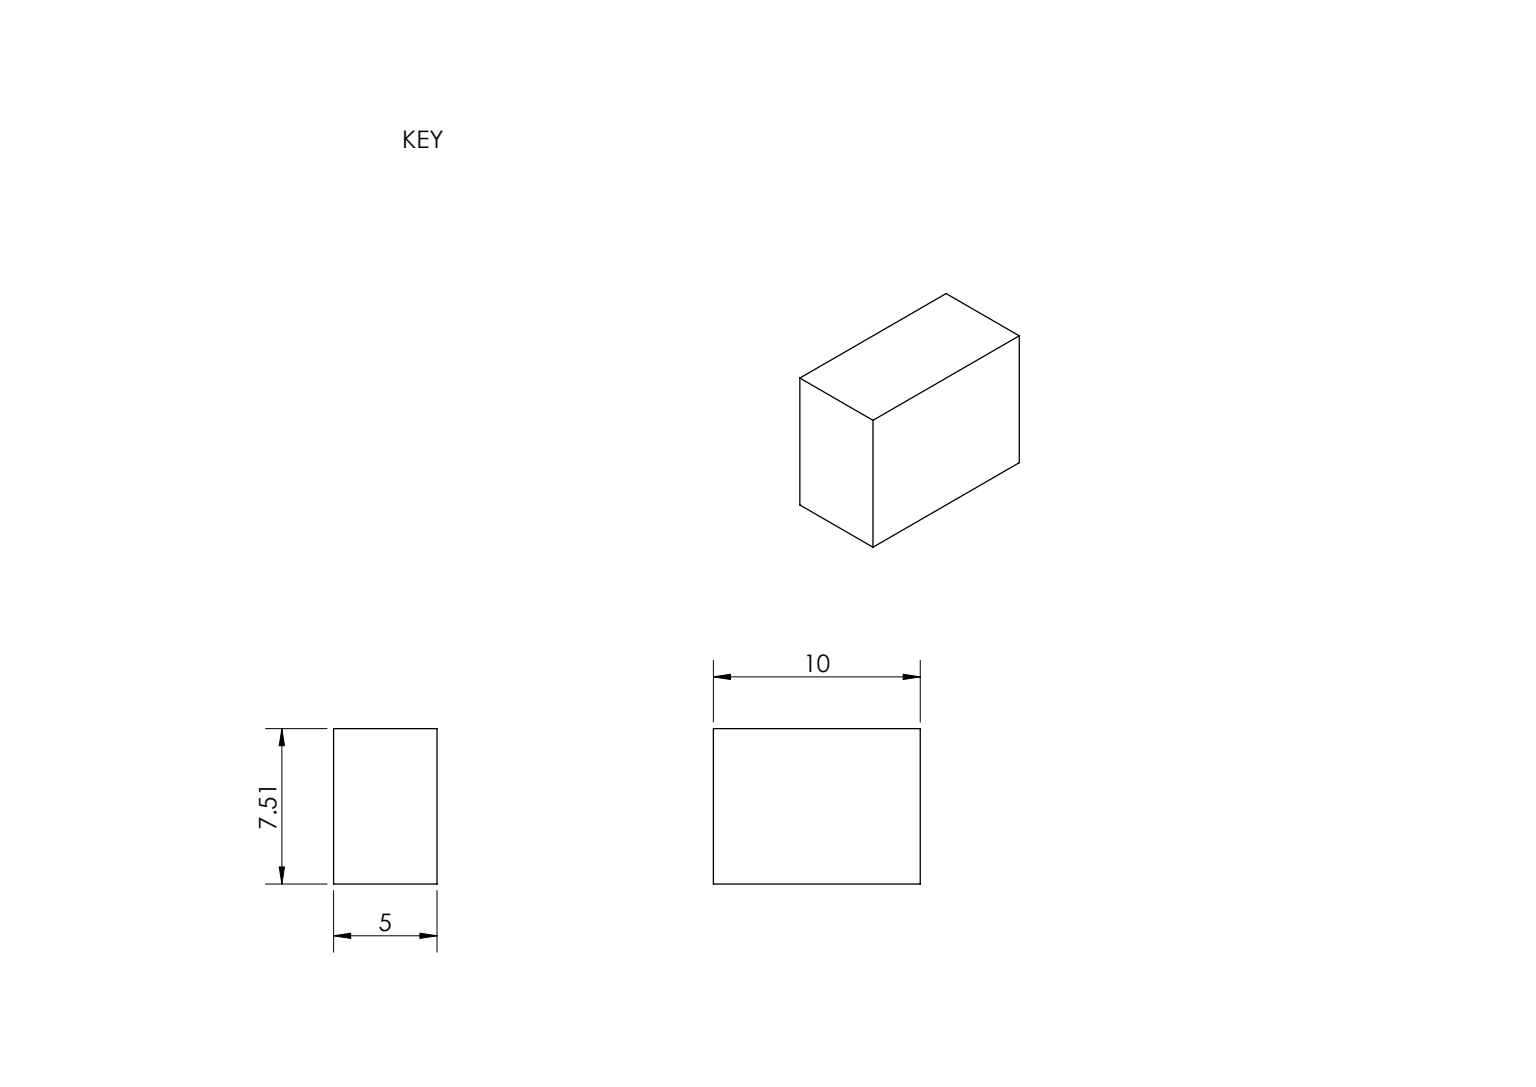
ISO-10303-21;
HEADER;
FILE_DESCRIPTION (('STEP AP214'),
    '1' );
FILE_NAME ('key.step',
    '2026-10-08T09:53:37',
    ( '' ),
    ( '' ),
    'SwSTEP 2.0',
    'SolidWorks 2026',
    '' );
FILE_SCHEMA (( 'AUTOMOTIVE_DESIGN' ));
ENDSEC;

DATA;
#19=AXIS2_PLACEMENT_3D ( 'NONE', #55225, #15366, #9737 ) ;
#383=( GEOMETRIC_REPRESENTATION_CONTEXT ( 3 ) GLOBAL_UNCERTAINTY_ASSIGNED_CONTEXT ( ( #16132 ) ) GLOBAL_UNIT_ASSIGNED_CONTEXT ( ( #58527, #47619, #18304 ) ) REPRESENTATION_CONTEXT ( 'NONE', 'WORKASPACE' ) );
#670=PLANE ( 'NONE',  #22865 ) ;
#687=ORIENTED_EDGE ( 'NONE', *, *, #21533, .F. ) ;
#692=SURFACE_SIDE_STYLE ('',( #30321 ) ) ;
#695=PLANE ( 'NONE',  #20980 ) ;
#1023=DIRECTION ( 'NONE',  ( 0.000000000000000000, -1.000000000000000000, 0.000000000000000000 ) ) ;
#1746=DIRECTION ( 'NONE',  ( -1.000000000000000000, -0.000000000000000000, -0.000000000000000000 ) ) ;
#2167=EDGE_CURVE ( 'NONE', #37724, #39945, #55632, .T. ) ;
#2801=DIRECTION ( 'NONE',  ( 0.000000000000000000, 1.000000000000000000, 0.000000000000000000 ) ) ;
#3898=VECTOR ( 'NONE', #1746, 1000.000000000000000 ) ;
#3952=MECHANICAL_DESIGN_GEOMETRIC_PRESENTATION_REPRESENTATION('',(#71150),#383);
#4204=( LENGTH_UNIT ( ) NAMED_UNIT ( * ) SI_UNIT ( .MILLI., .METRE. ) );
#4518=EDGE_CURVE ( 'NONE', #39945, #5325, #48483, .T. ) ;
#4952=SURFACE_SIDE_STYLE ('',( #9080 ) ) ;
#5325=VERTEX_POINT ( 'NONE', #24542 ) ;
#6306=( NAMED_UNIT ( * ) SI_UNIT ( $, .STERADIAN. ) SOLID_ANGLE_UNIT ( ) );
#6406=PRODUCT_DEFINITION_FORMATION_WITH_SPECIFIED_SOURCE ( 'ANY', '', #48755, .NOT_KNOWN. ) ;
#6637=FACE_OUTER_BOUND ( 'NONE', #63194, .T. ) ;
#6650=CARTESIAN_POINT ( 'NONE',  ( -2.499999999999997780, 8.494897427831771708, -19.01812422950394676 ) ) ;
#6662=SURFACE_STYLE_USAGE ( .BOTH. , #692 ) ;
#6695=VERTEX_POINT ( 'NONE', #45004 ) ;
#8097=DIRECTION ( 'NONE',  ( 0.000000000000000000, -0.000000000000000000, -1.000000000000000000 ) ) ;
#9080=SURFACE_STYLE_FILL_AREA ( #72225 ) ;
#9224=EDGE_CURVE ( 'NONE', #34982, #38545, #28058, .T. ) ;
#9388=CARTESIAN_POINT ( 'NONE',  ( -2.500000000000000000, 16.00000000000000000, 0.000000000000000000 ) ) ;
#9609=EDGE_CURVE ( 'NONE', #5325, #55639, #73082, .T. ) ;
#9737=DIRECTION ( 'NONE',  ( 2.889240119132116694E-16, -1.000000000000000000, 0.000000000000000000 ) ) ;
#9969=APPLICATION_CONTEXT ( 'automotive_design' ) ;
#10321=CARTESIAN_POINT ( 'NONE',  ( -2.500000000000000000, 16.00000000000000000, -10.00000000000000178 ) ) ;
#11069=EDGE_CURVE ( 'NONE', #6695, #34982, #20563, .T. ) ;
#11908=LINE ( 'NONE', #6650, #41232 ) ;
#11959=ORIENTED_EDGE ( 'NONE', *, *, #63581, .T. ) ;
#12006=DIRECTION ( 'NONE',  ( -0.000000000000000000, 0.000000000000000000, 1.000000000000000000 ) ) ;
#14915=DIRECTION ( 'NONE',  ( 5.778480238264233142E-17, -1.000000000000000000, 0.000000000000000000 ) ) ;
#14998=FACE_OUTER_BOUND ( 'NONE', #61959, .T. ) ;
#15064=ORIENTED_EDGE ( 'NONE', *, *, #72245, .F. ) ;
#15098=ORIENTED_EDGE ( 'NONE', *, *, #11069, .T. ) ;
#15366=DIRECTION ( 'NONE',  ( -1.000000000000000000, -2.889240119132116694E-16, 0.000000000000000000 ) ) ;
#15700=EDGE_CURVE ( 'NONE', #38545, #39945, #11908, .T. ) ;
#16132=UNCERTAINTY_MEASURE_WITH_UNIT (LENGTH_MEASURE( 1.000000000000000082E-05 ), #58527, 'distance_accuracy_value', 'NONE');
#16180=LINE ( 'NONE', #21069, #61063 ) ;
#16797=CARTESIAN_POINT ( 'NONE',  ( -2.499999999999997780, 8.494897427831771708, -10.00000000000000178 ) ) ;
#17069=ORIENTED_EDGE ( 'NONE', *, *, #36059, .T. ) ;
#17917=DIRECTION ( 'NONE',  ( 1.000000000000000000, 5.778480238264233142E-17, -0.000000000000000000 ) ) ;
#17942=FILL_AREA_STYLE_COLOUR ( '', #26671 ) ;
#18292=CARTESIAN_POINT ( 'NONE',  ( -2.499999999999997780, 8.494897427831771708, -10.00000000000000178 ) ) ;
#18304=( NAMED_UNIT ( * ) SI_UNIT ( $, .STERADIAN. ) SOLID_ANGLE_UNIT ( ) );
#18325=LINE ( 'NONE', #52532, #45553 ) ;
#18875=DIRECTION ( 'NONE',  ( 0.000000000000000000, 0.000000000000000000, 1.000000000000000000 ) ) ;
#19089=DIRECTION ( 'NONE',  ( 0.000000000000000000, 0.000000000000000000, 1.000000000000000000 ) ) ;
#19252=CARTESIAN_POINT ( 'NONE',  ( 2.500000000000000000, 16.00000000000000000, -19.01812422950394676 ) ) ;
#19415=ADVANCED_FACE ( 'NONE', ( #45123 ), #28926, .T. ) ;
#19713=EDGE_LOOP ( 'NONE', ( #45893, #58178, #43286, #25168 ) ) ;
#19735=DIRECTION ( 'NONE',  ( 1.000000000000000000, 0.000000000000000000, 0.000000000000000000 ) ) ;
#20563=LINE ( 'NONE', #54042, #32379 ) ;
#20980=AXIS2_PLACEMENT_3D ( 'NONE', #23585, #23963, #69442 ) ;
#21069=CARTESIAN_POINT ( 'NONE',  ( -2.500000000000000000, 16.00000000000000000, -10.00000000000000178 ) ) ;
#21087=SURFACE_STYLE_USAGE ( .BOTH. , #4952 ) ;
#21154=PRODUCT_DEFINITION_SHAPE ( 'NONE', 'NONE',  #40301 ) ;
#21533=EDGE_CURVE ( 'NONE', #55639, #37724, #40538, .T. ) ;
#22865=AXIS2_PLACEMENT_3D ( 'NONE', #23558, #17917, #40861 ) ;
#23457=SHAPE_REPRESENTATION ( 'key', ( #43395 ), #59100 ) ;
#23558=CARTESIAN_POINT ( 'NONE',  ( 2.500000000000000000, 16.00000000000000000, -19.01812422950394676 ) ) ;
#23585=CARTESIAN_POINT ( 'NONE',  ( -1.066668064568189757E-15, -1.540743955509788682E-30, -10.00000000000000178 ) ) ;
#23963=DIRECTION ( 'NONE',  ( 0.000000000000000000, 0.000000000000000000, 1.000000000000000000 ) ) ;
#24542=CARTESIAN_POINT ( 'NONE',  ( 2.500000000000000444, 8.494897427831771708, 0.000000000000000000 ) ) ;
#24637=ORIENTED_EDGE ( 'NONE', *, *, #4518, .F. ) ;
#25168=ORIENTED_EDGE ( 'NONE', *, *, #21533, .T. ) ;
#25559=ADVANCED_FACE ( 'NONE', ( #57806 ), #695, .F. ) ;
#26299=( GEOMETRIC_REPRESENTATION_CONTEXT ( 3 ) GLOBAL_UNCERTAINTY_ASSIGNED_CONTEXT ( ( #43771 ) ) GLOBAL_UNIT_ASSIGNED_CONTEXT ( ( #4204, #50028, #27096 ) ) REPRESENTATION_CONTEXT ( 'NONE', 'WORKASPACE' ) );
#26312=DIRECTION ( 'NONE',  ( 2.889240119132116694E-16, -1.000000000000000000, 0.000000000000000000 ) ) ;
#26611=VECTOR ( 'NONE', #65778, 1000.000000000000000 ) ;
#26671=COLOUR_RGB ( '', 0.66274510, 0.83137255, 0.94901961) ;
#27096=( NAMED_UNIT ( * ) SI_UNIT ( $, .STERADIAN. ) SOLID_ANGLE_UNIT ( ) );
#27153=ORIENTED_EDGE ( 'NONE', *, *, #11069, .F. ) ;
#28058=LINE ( 'NONE', #16797, #52879 ) ;
#28545=CARTESIAN_POINT ( 'NONE',  ( 0.000000000000000000, 0.000000000000000000, 0.000000000000000000 ) ) ;
#28600=CARTESIAN_POINT ( 'NONE',  ( 2.500000000000000000, 16.00000000000000000, 0.000000000000000000 ) ) ;
#28926=PLANE ( 'NONE',  #49773 ) ;
#29703=ADVANCED_FACE ( 'NONE', ( #29908 ), #48322, .T. ) ;
#29908=FACE_OUTER_BOUND ( 'NONE', #35122, .T. ) ;
#30321=SURFACE_STYLE_FILL_AREA ( #52147 ) ;
#30386=VECTOR ( 'NONE', #19089, 1000.000000000000000 ) ;
#30580=PLANE ( 'NONE',  #43045 ) ;
#31609=CARTESIAN_POINT ( 'NONE',  ( -2.499999999999997780, 8.494897427831771708, 0.000000000000000000 ) ) ;
#32283=PLANE ( 'NONE',  #19 ) ;
#32379=VECTOR ( 'NONE', #14915, 1000.000000000000000 ) ;
#32504=ADVANCED_FACE ( 'NONE', ( #66299 ), #30580, .T. ) ;
#33333=ORIENTED_EDGE ( 'NONE', *, *, #2167, .F. ) ;
#34866=( NAMED_UNIT ( * ) PLANE_ANGLE_UNIT ( ) SI_UNIT ( $, .RADIAN. ) );
#34982=VERTEX_POINT ( 'NONE', #65531 ) ;
#35122=EDGE_LOOP ( 'NONE', ( #69723, #38672, #24637, #71523 ) ) ;
#35908=STYLED_ITEM ( 'NONE', ( #45160 ), #63624 ) ;
#36059=EDGE_CURVE ( 'NONE', #38545, #50675, #57683, .T. ) ;
#36243=EDGE_LOOP ( 'NONE', ( #69673, #54921, #687, #38370 ) ) ;
#37724=VERTEX_POINT ( 'NONE', #68878 ) ;
#37754=UNCERTAINTY_MEASURE_WITH_UNIT (LENGTH_MEASURE( 1.000000000000000082E-05 ), #47260, 'distance_accuracy_value', 'NONE');
#38370=ORIENTED_EDGE ( 'NONE', *, *, #63581, .F. ) ;
#38545=VERTEX_POINT ( 'NONE', #18292 ) ;
#38672=ORIENTED_EDGE ( 'NONE', *, *, #72245, .T. ) ;
#39643=CARTESIAN_POINT ( 'NONE',  ( -2.500000000000000000, 16.00000000000000000, -10.00000000000000178 ) ) ;
#39829=VECTOR ( 'NONE', #26312, 1000.000000000000000 ) ;
#39945=VERTEX_POINT ( 'NONE', #31609 ) ;
#39953=EDGE_CURVE ( 'NONE', #50675, #6695, #16180, .T. ) ;
#40301=PRODUCT_DEFINITION ( 'UNKNOWN', '', #6406, #54422 ) ;
#40538=LINE ( 'NONE', #63485, #3898 ) ;
#40737=APPLICATION_CONTEXT ( 'automotive_design' ) ;
#40849=CARTESIAN_POINT ( 'NONE',  ( -2.499999999999997780, 8.494897427831771708, -19.01812422950394676 ) ) ;
#40861=DIRECTION ( 'NONE',  ( -5.778480238264233142E-17, 1.000000000000000000, 0.000000000000000000 ) ) ;
#41232=VECTOR ( 'NONE', #63809, 1000.000000000000000 ) ;
#41608=SHAPE_REPRESENTATION_RELATIONSHIP ( 'NONE' , 'NONE' ,  #23457, #55235 ) ;
#42783=CLOSED_SHELL ( 'NONE', ( #64028, #32504, #45108, #29703, #19415, #25559 ) ) ;
#43045=AXIS2_PLACEMENT_3D ( 'NONE', #60657, #2801, #60295 ) ;
#43286=ORIENTED_EDGE ( 'NONE', *, *, #9609, .T. ) ;
#43395=AXIS2_PLACEMENT_3D ( 'NONE', #48320, #71232, #19735 ) ;
#43661=DIRECTION ( 'NONE',  ( 1.000000000000000000, 0.000000000000000000, 0.000000000000000000 ) ) ;
#43703=ORIENTED_EDGE ( 'NONE', *, *, #15700, .T. ) ;
#43771=UNCERTAINTY_MEASURE_WITH_UNIT (LENGTH_MEASURE( 1.000000000000000082E-05 ), #4204, 'distance_accuracy_value', 'NONE');
#45004=CARTESIAN_POINT ( 'NONE',  ( 2.500000000000000000, 16.00000000000000000, -10.00000000000000178 ) ) ;
#45108=ADVANCED_FACE ( 'NONE', ( #6637 ), #670, .T. ) ;
#45123=FACE_OUTER_BOUND ( 'NONE', #19713, .T. ) ;
#45160=PRESENTATION_STYLE_ASSIGNMENT (( #21087 ) ) ;
#45553=VECTOR ( 'NONE', #59295, 1000.000000000000000 ) ;
#45666=DIRECTION ( 'NONE',  ( -5.778480238264233142E-17, 1.000000000000000000, -0.000000000000000000 ) ) ;
#45671=DIRECTION ( 'NONE',  ( -2.889240119132116694E-16, 1.000000000000000000, 0.000000000000000000 ) ) ;
#45877=DIRECTION ( 'NONE',  ( 1.000000000000000000, 0.000000000000000000, 0.000000000000000000 ) ) ;
#45893=ORIENTED_EDGE ( 'NONE', *, *, #2167, .T. ) ;
#47055=VECTOR ( 'NONE', #45671, 1000.000000000000000 ) ;
#47260=( LENGTH_UNIT ( ) NAMED_UNIT ( * ) SI_UNIT ( .MILLI., .METRE. ) );
#47619=( NAMED_UNIT ( * ) PLANE_ANGLE_UNIT ( ) SI_UNIT ( $, .RADIAN. ) );
#47937=COLOUR_RGB ( '', 0.66274510, 0.83137255, 0.94901961) ;
#48320=CARTESIAN_POINT ( 'NONE',  ( 0.000000000000000000, 0.000000000000000000, 0.000000000000000000 ) ) ;
#48322=PLANE ( 'NONE',  #69402 ) ;
#48483=LINE ( 'NONE', #71398, #26611 ) ;
#48755=PRODUCT ( 'key', 'key', '', ( #66680 ) ) ;
#48963=ORIENTED_EDGE ( 'NONE', *, *, #56177, .F. ) ;
#49108=MECHANICAL_DESIGN_GEOMETRIC_PRESENTATION_REPRESENTATION('',(#35908),#26299);
#49773=AXIS2_PLACEMENT_3D ( 'NONE', #28545, #12006, #45877 ) ;
#50028=( NAMED_UNIT ( * ) PLANE_ANGLE_UNIT ( ) SI_UNIT ( $, .RADIAN. ) );
#50253=VECTOR ( 'NONE', #45666, 1000.000000000000000 ) ;
#50675=VERTEX_POINT ( 'NONE', #39643 ) ;
#52147=FILL_AREA_STYLE ('',( #17942 ) ) ;
#52532=CARTESIAN_POINT ( 'NONE',  ( 2.500000000000000444, 8.494897427831771708, -19.01812422950394676 ) ) ;
#52879=VECTOR ( 'NONE', #63402, 1000.000000000000000 ) ;
#53676=LINE ( 'NONE', #59695, #30386 ) ;
#54042=CARTESIAN_POINT ( 'NONE',  ( 2.500000000000000000, 16.00000000000000000, -10.00000000000000178 ) ) ;
#54422=PRODUCT_DEFINITION_CONTEXT ( 'detailed design', #40737, 'design' ) ;
#54921=ORIENTED_EDGE ( 'NONE', *, *, #56177, .T. ) ;
#55225=CARTESIAN_POINT ( 'NONE',  ( -2.500000000000000000, 16.00000000000000000, -19.01812422950394676 ) ) ;
#55235=ADVANCED_BREP_SHAPE_REPRESENTATION ( '', ( #63624, #43395 ), #59100 ) ;
#55632=LINE ( 'NONE', #9388, #39829 ) ;
#55639=VERTEX_POINT ( 'NONE', #28600 ) ;
#56177=EDGE_CURVE ( 'NONE', #50675, #37724, #53676, .T. ) ;
#56182=CARTESIAN_POINT ( 'NONE',  ( 2.500000000000000000, 16.00000000000000000, 0.000000000000000000 ) ) ;
#56891=SHAPE_DEFINITION_REPRESENTATION ( #21154, #23457 ) ;
#57328=ORIENTED_EDGE ( 'NONE', *, *, #39953, .T. ) ;
#57683=LINE ( 'NONE', #10321, #47055 ) ;
#57806=FACE_OUTER_BOUND ( 'NONE', #65461, .T. ) ;
#58178=ORIENTED_EDGE ( 'NONE', *, *, #4518, .T. ) ;
#58527=( LENGTH_UNIT ( ) NAMED_UNIT ( * ) SI_UNIT ( .MILLI., .METRE. ) );
#59100=( GEOMETRIC_REPRESENTATION_CONTEXT ( 3 ) GLOBAL_UNCERTAINTY_ASSIGNED_CONTEXT ( ( #37754 ) ) GLOBAL_UNIT_ASSIGNED_CONTEXT ( ( #47260, #34866, #6306 ) ) REPRESENTATION_CONTEXT ( 'NONE', 'WORKASPACE' ) );
#59295=DIRECTION ( 'NONE',  ( 0.000000000000000000, 0.000000000000000000, 1.000000000000000000 ) ) ;
#59339=ORIENTED_EDGE ( 'NONE', *, *, #36059, .F. ) ;
#59695=CARTESIAN_POINT ( 'NONE',  ( -2.500000000000000000, 16.00000000000000000, -19.01812422950394676 ) ) ;
#59843=ORIENTED_EDGE ( 'NONE', *, *, #9609, .F. ) ;
#60295=DIRECTION ( 'NONE',  ( 0.000000000000000000, -0.000000000000000000, 1.000000000000000000 ) ) ;
#60657=CARTESIAN_POINT ( 'NONE',  ( -2.500000000000000000, 16.00000000000000000, -19.01812422950394676 ) ) ;
#61063=VECTOR ( 'NONE', #43661, 1000.000000000000000 ) ;
#61959=EDGE_LOOP ( 'NONE', ( #59339, #43703, #33333, #48963 ) ) ;
#63194=EDGE_LOOP ( 'NONE', ( #27153, #11959, #59843, #15064 ) ) ;
#63402=DIRECTION ( 'NONE',  ( -1.000000000000000000, 0.000000000000000000, 0.000000000000000000 ) ) ;
#63485=CARTESIAN_POINT ( 'NONE',  ( -2.500000000000000000, 16.00000000000000000, 0.000000000000000000 ) ) ;
#63581=EDGE_CURVE ( 'NONE', #6695, #55639, #71849, .T. ) ;
#63624=MANIFOLD_SOLID_BREP ( 'Boss-Extrude1', #42783 ) ;
#63809=DIRECTION ( 'NONE',  ( 0.000000000000000000, 0.000000000000000000, 1.000000000000000000 ) ) ;
#64028=ADVANCED_FACE ( 'NONE', ( #14998 ), #32283, .T. ) ;
#64928=PRESENTATION_STYLE_ASSIGNMENT (( #6662 ) ) ;
#65461=EDGE_LOOP ( 'NONE', ( #17069, #57328, #15098, #70522 ) ) ;
#65531=CARTESIAN_POINT ( 'NONE',  ( 2.500000000000000444, 8.494897427831771708, -10.00000000000000178 ) ) ;
#65778=DIRECTION ( 'NONE',  ( 1.000000000000000000, 0.000000000000000000, 0.000000000000000000 ) ) ;
#66299=FACE_OUTER_BOUND ( 'NONE', #36243, .T. ) ;
#66680=PRODUCT_CONTEXT ( 'NONE', #9969, 'mechanical' ) ;
#67145=VECTOR ( 'NONE', #18875, 1000.000000000000000 ) ;
#67713=FILL_AREA_STYLE_COLOUR ( '', #47937 ) ;
#68878=CARTESIAN_POINT ( 'NONE',  ( -2.500000000000000000, 16.00000000000000000, 0.000000000000000000 ) ) ;
#69402=AXIS2_PLACEMENT_3D ( 'NONE', #40849, #1023, #8097 ) ;
#69442=DIRECTION ( 'NONE',  ( 1.000000000000000000, 0.000000000000000000, 0.000000000000000000 ) ) ;
#69673=ORIENTED_EDGE ( 'NONE', *, *, #39953, .F. ) ;
#69723=ORIENTED_EDGE ( 'NONE', *, *, #9224, .F. ) ;
#70522=ORIENTED_EDGE ( 'NONE', *, *, #9224, .T. ) ;
#71150=STYLED_ITEM ( 'NONE', ( #64928 ), #55235 ) ;
#71232=DIRECTION ( 'NONE',  ( 0.000000000000000000, 0.000000000000000000, 1.000000000000000000 ) ) ;
#71398=CARTESIAN_POINT ( 'NONE',  ( -2.499999999999997780, 8.494897427831771708, 0.000000000000000000 ) ) ;
#71523=ORIENTED_EDGE ( 'NONE', *, *, #15700, .F. ) ;
#71849=LINE ( 'NONE', #19252, #67145 ) ;
#72225=FILL_AREA_STYLE ('',( #67713 ) ) ;
#72245=EDGE_CURVE ( 'NONE', #34982, #5325, #18325, .T. ) ;
#73082=LINE ( 'NONE', #56182, #50253 ) ;
ENDSEC;
END-ISO-10303-21;
